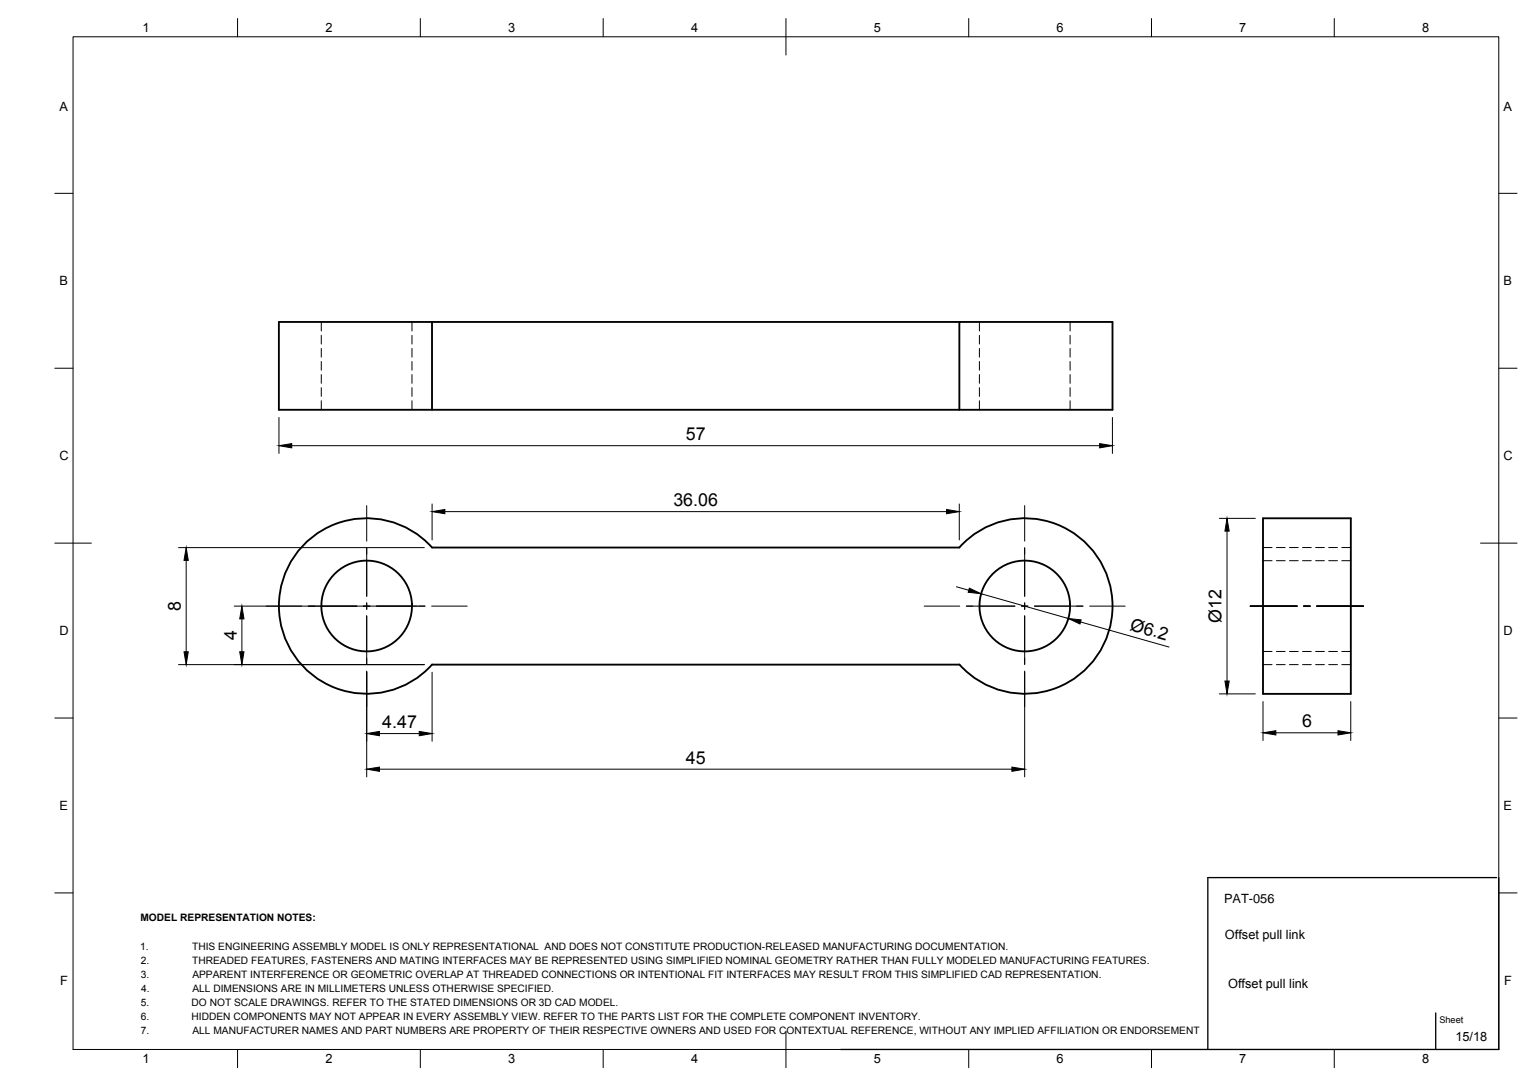
ISO-10303-21;
HEADER;
/* Generated by software containing ST-Developer
 * from STEP Tools, Inc. (www.steptools.com) 
 */

FILE_DESCRIPTION(
/* description */ ('Hook toggle clamp'),
/* implementation_level */ '2;1');

FILE_NAME(
/* name */ 'Offset pull link.step',
/* time_stamp */ '2026-10-27T21:56:56-07:00',
/* author */ (''),
/* organization */ (''),
/* preprocessor_version */ 'ST-DEVELOPER v20.2',
/* originating_system */ 'Autodesk Translation Framework v15.17.0.0',
/* authorisation */ '');

FILE_SCHEMA (('AUTOMOTIVE_DESIGN { 1 0 10303 214 3 1 1 }'));
ENDSEC;

DATA;
#10=MECHANICAL_DESIGN_GEOMETRIC_PRESENTATION_REPRESENTATION('',(#197),#5458);
#163=SHAPE_REPRESENTATION_RELATIONSHIP('SRR','None',#5546,#180);
#180=ADVANCED_BREP_SHAPE_REPRESENTATION('',(#213),#5448);
#197=STYLED_ITEM('',(#5703),#213);
#213=MANIFOLD_SOLID_BREP('Body1',#2979);
#255=FACE_BOUND('',#707,.T.);
#256=FACE_BOUND('',#708,.T.);
#257=FACE_BOUND('',#712,.T.);
#258=FACE_BOUND('',#713,.T.);
#352=PLANE('',#3359);
#353=PLANE('',#3360);
#354=PLANE('',#3362);
#355=PLANE('',#3365);
#496=FACE_OUTER_BOUND('',#702,.T.);
#497=FACE_OUTER_BOUND('',#703,.T.);
#498=FACE_OUTER_BOUND('',#704,.T.);
#499=FACE_OUTER_BOUND('',#705,.T.);
#500=FACE_OUTER_BOUND('',#706,.T.);
#501=FACE_OUTER_BOUND('',#709,.T.);
#502=FACE_OUTER_BOUND('',#710,.T.);
#503=FACE_OUTER_BOUND('',#711,.T.);
#702=EDGE_LOOP('',(#2461,#2462,#2463,#2464));
#703=EDGE_LOOP('',(#2465,#2466,#2467,#2468));
#704=EDGE_LOOP('',(#2469,#2470,#2471,#2472));
#705=EDGE_LOOP('',(#2473,#2474,#2475,#2476));
#706=EDGE_LOOP('',(#2477,#2478,#2479,#2480));
#707=EDGE_LOOP('',(#2481));
#708=EDGE_LOOP('',(#2482));
#709=EDGE_LOOP('',(#2483,#2484,#2485,#2486));
#710=EDGE_LOOP('',(#2487,#2488,#2489,#2490));
#711=EDGE_LOOP('',(#2491,#2492,#2493,#2494));
#712=EDGE_LOOP('',(#2495));
#713=EDGE_LOOP('',(#2496));
#961=LINE('',#4932,#1198);
#962=LINE('',#4938,#1199);
#963=LINE('',#4943,#1200);
#964=LINE('',#4947,#1201);
#965=LINE('',#4951,#1202);
#966=LINE('',#4953,#1203);
#967=LINE('',#4954,#1204);
#968=LINE('',#4957,#1205);
#969=LINE('',#4961,#1206);
#970=LINE('',#4962,#1207);
#1198=VECTOR('',#4029,0.31);
#1199=VECTOR('',#4036,0.31);
#1200=VECTOR('',#4041,1.);
#1201=VECTOR('',#4044,1.);
#1202=VECTOR('',#4049,1.);
#1203=VECTOR('',#4050,1.);
#1204=VECTOR('',#4051,1.);
#1205=VECTOR('',#4054,1.);
#1206=VECTOR('',#4059,1.);
#1207=VECTOR('',#4060,1.);
#1327=CIRCLE('',#3351,0.31);
#1328=CIRCLE('',#3352,0.31);
#1329=CIRCLE('',#3354,0.31);
#1330=CIRCLE('',#3355,0.31);
#1331=CIRCLE('',#3357,0.6);
#1332=CIRCLE('',#3358,0.6);
#1333=CIRCLE('',#3361,0.6);
#1334=CIRCLE('',#3364,0.6);
#1534=VERTEX_POINT('',#4929);
#1535=VERTEX_POINT('',#4931);
#1536=VERTEX_POINT('',#4935);
#1537=VERTEX_POINT('',#4937);
#1538=VERTEX_POINT('',#4941);
#1539=VERTEX_POINT('',#4942);
#1540=VERTEX_POINT('',#4944);
#1541=VERTEX_POINT('',#4946);
#1542=VERTEX_POINT('',#4950);
#1543=VERTEX_POINT('',#4952);
#1544=VERTEX_POINT('',#4956);
#1545=VERTEX_POINT('',#4960);
#1857=EDGE_CURVE('',#1534,#1534,#1327,.T.);
#1858=EDGE_CURVE('',#1534,#1535,#961,.T.);
#1859=EDGE_CURVE('',#1535,#1535,#1328,.T.);
#1860=EDGE_CURVE('',#1536,#1536,#1329,.T.);
#1861=EDGE_CURVE('',#1536,#1537,#962,.T.);
#1862=EDGE_CURVE('',#1537,#1537,#1330,.T.);
#1863=EDGE_CURVE('',#1538,#1539,#963,.T.);
#1864=EDGE_CURVE('',#1540,#1538,#1331,.T.);
#1865=EDGE_CURVE('',#1541,#1540,#964,.T.);
#1866=EDGE_CURVE('',#1541,#1539,#1332,.T.);
#1867=EDGE_CURVE('',#1539,#1542,#965,.T.);
#1868=EDGE_CURVE('',#1543,#1542,#966,.T.);
#1869=EDGE_CURVE('',#1538,#1543,#967,.T.);
#1870=EDGE_CURVE('',#1544,#1541,#968,.T.);
#1871=EDGE_CURVE('',#1542,#1544,#1333,.T.);
#1872=EDGE_CURVE('',#1545,#1540,#969,.T.);
#1873=EDGE_CURVE('',#1544,#1545,#970,.T.);
#1874=EDGE_CURVE('',#1543,#1545,#1334,.T.);
#2461=ORIENTED_EDGE('',*,*,#1857,.F.);
#2462=ORIENTED_EDGE('',*,*,#1858,.T.);
#2463=ORIENTED_EDGE('',*,*,#1859,.F.);
#2464=ORIENTED_EDGE('',*,*,#1858,.F.);
#2465=ORIENTED_EDGE('',*,*,#1860,.F.);
#2466=ORIENTED_EDGE('',*,*,#1861,.T.);
#2467=ORIENTED_EDGE('',*,*,#1862,.F.);
#2468=ORIENTED_EDGE('',*,*,#1861,.F.);
#2469=ORIENTED_EDGE('',*,*,#1863,.F.);
#2470=ORIENTED_EDGE('',*,*,#1864,.F.);
#2471=ORIENTED_EDGE('',*,*,#1865,.F.);
#2472=ORIENTED_EDGE('',*,*,#1866,.T.);
#2473=ORIENTED_EDGE('',*,*,#1863,.T.);
#2474=ORIENTED_EDGE('',*,*,#1867,.T.);
#2475=ORIENTED_EDGE('',*,*,#1868,.F.);
#2476=ORIENTED_EDGE('',*,*,#1869,.F.);
#2477=ORIENTED_EDGE('',*,*,#1866,.F.);
#2478=ORIENTED_EDGE('',*,*,#1870,.F.);
#2479=ORIENTED_EDGE('',*,*,#1871,.F.);
#2480=ORIENTED_EDGE('',*,*,#1867,.F.);
#2481=ORIENTED_EDGE('',*,*,#1857,.T.);
#2482=ORIENTED_EDGE('',*,*,#1860,.T.);
#2483=ORIENTED_EDGE('',*,*,#1865,.T.);
#2484=ORIENTED_EDGE('',*,*,#1872,.F.);
#2485=ORIENTED_EDGE('',*,*,#1873,.F.);
#2486=ORIENTED_EDGE('',*,*,#1870,.T.);
#2487=ORIENTED_EDGE('',*,*,#1868,.T.);
#2488=ORIENTED_EDGE('',*,*,#1871,.T.);
#2489=ORIENTED_EDGE('',*,*,#1873,.T.);
#2490=ORIENTED_EDGE('',*,*,#1874,.F.);
#2491=ORIENTED_EDGE('',*,*,#1869,.T.);
#2492=ORIENTED_EDGE('',*,*,#1874,.T.);
#2493=ORIENTED_EDGE('',*,*,#1872,.T.);
#2494=ORIENTED_EDGE('',*,*,#1864,.T.);
#2495=ORIENTED_EDGE('',*,*,#1859,.T.);
#2496=ORIENTED_EDGE('',*,*,#1862,.T.);
#2774=CYLINDRICAL_SURFACE('',#3350,0.31);
#2775=CYLINDRICAL_SURFACE('',#3353,0.31);
#2776=CYLINDRICAL_SURFACE('',#3356,0.6);
#2777=CYLINDRICAL_SURFACE('',#3363,0.6);
#2900=ADVANCED_FACE('',(#496),#2774,.F.);
#2901=ADVANCED_FACE('',(#497),#2775,.F.);
#2902=ADVANCED_FACE('',(#498),#2776,.T.);
#2903=ADVANCED_FACE('',(#499),#352,.T.);
#2904=ADVANCED_FACE('',(#500,#255,#256),#353,.F.);
#2905=ADVANCED_FACE('',(#501),#354,.T.);
#2906=ADVANCED_FACE('',(#502),#2777,.T.);
#2907=ADVANCED_FACE('',(#503,#257,#258),#355,.T.);
#2979=CLOSED_SHELL('',(#2900,#2901,#2902,#2903,#2904,#2905,#2906,#2907));
#3349=AXIS2_PLACEMENT_3D('',#4927,#4023,#4024);
#3350=AXIS2_PLACEMENT_3D('',#4928,#4025,#4026);
#3351=AXIS2_PLACEMENT_3D('',#4930,#4027,#4028);
#3352=AXIS2_PLACEMENT_3D('',#4933,#4030,#4031);
#3353=AXIS2_PLACEMENT_3D('',#4934,#4032,#4033);
#3354=AXIS2_PLACEMENT_3D('',#4936,#4034,#4035);
#3355=AXIS2_PLACEMENT_3D('',#4939,#4037,#4038);
#3356=AXIS2_PLACEMENT_3D('',#4940,#4039,#4040);
#3357=AXIS2_PLACEMENT_3D('',#4945,#4042,#4043);
#3358=AXIS2_PLACEMENT_3D('',#4948,#4045,#4046);
#3359=AXIS2_PLACEMENT_3D('',#4949,#4047,#4048);
#3360=AXIS2_PLACEMENT_3D('',#4955,#4052,#4053);
#3361=AXIS2_PLACEMENT_3D('',#4958,#4055,#4056);
#3362=AXIS2_PLACEMENT_3D('',#4959,#4057,#4058);
#3363=AXIS2_PLACEMENT_3D('',#4963,#4061,#4062);
#3364=AXIS2_PLACEMENT_3D('',#4964,#4063,#4064);
#3365=AXIS2_PLACEMENT_3D('',#4965,#4065,#4066);
#4023=DIRECTION('axis',(0.,0.,1.));
#4024=DIRECTION('refdir',(1.,0.,0.));
#4025=DIRECTION('center_axis',(0.,1.,0.));
#4026=DIRECTION('ref_axis',(1.,0.,0.));
#4027=DIRECTION('center_axis',(0.,1.,0.));
#4028=DIRECTION('ref_axis',(1.,0.,0.));
#4029=DIRECTION('',(0.,1.,0.));
#4030=DIRECTION('center_axis',(0.,-1.,0.));
#4031=DIRECTION('ref_axis',(1.,0.,0.));
#4032=DIRECTION('center_axis',(0.,1.,0.));
#4033=DIRECTION('ref_axis',(1.,0.,0.));
#4034=DIRECTION('center_axis',(0.,1.,0.));
#4035=DIRECTION('ref_axis',(1.,0.,0.));
#4036=DIRECTION('',(0.,1.,0.));
#4037=DIRECTION('center_axis',(0.,-1.,0.));
#4038=DIRECTION('ref_axis',(1.,0.,0.));
#4039=DIRECTION('center_axis',(0.,1.,0.));
#4040=DIRECTION('ref_axis',(1.,0.,0.));
#4041=DIRECTION('',(0.,-1.,0.));
#4042=DIRECTION('center_axis',(0.,1.,0.));
#4043=DIRECTION('ref_axis',(1.,0.,0.));
#4044=DIRECTION('',(0.,1.,0.));
#4045=DIRECTION('center_axis',(0.,1.,0.));
#4046=DIRECTION('ref_axis',(1.,0.,0.));
#4047=DIRECTION('center_axis',(0.0484198570820323,0.,-0.998827070838669));
#4048=DIRECTION('ref_axis',(-0.998827070838669,0.,-0.0484198570820323));
#4049=DIRECTION('',(-0.998827070838669,0.,-0.0484198570820323));
#4050=DIRECTION('',(0.,-1.,0.));
#4051=DIRECTION('',(-0.998827070838669,0.,-0.0484198570820323));
#4052=DIRECTION('center_axis',(0.,1.,0.));
#4053=DIRECTION('ref_axis',(1.,0.,0.));
#4054=DIRECTION('',(0.998827070838669,0.,0.0484198570820322));
#4055=DIRECTION('center_axis',(0.,1.,0.));
#4056=DIRECTION('ref_axis',(1.,0.,0.));
#4057=DIRECTION('center_axis',(-0.0484198570820322,0.,0.998827070838669));
#4058=DIRECTION('ref_axis',(0.998827070838669,0.,0.0484198570820322));
#4059=DIRECTION('',(0.998827070838669,0.,0.0484198570820322));
#4060=DIRECTION('',(0.,1.,0.));
#4061=DIRECTION('center_axis',(0.,1.,0.));
#4062=DIRECTION('ref_axis',(-0.998827070838669,0.,-0.0484198570820321));
#4063=DIRECTION('center_axis',(0.,1.,0.));
#4064=DIRECTION('ref_axis',(1.,0.,0.));
#4065=DIRECTION('center_axis',(0.,1.,0.));
#4066=DIRECTION('ref_axis',(1.,0.,0.));
#4927=CARTESIAN_POINT('',(0.,0.,0.));
#4928=CARTESIAN_POINT('Origin',(-2.49048674522936,1.,2.28211064313086));
#4929=CARTESIAN_POINT('',(-2.80048674522936,1.1,2.28211064313086));
#4930=CARTESIAN_POINT('Origin',(-2.49048674522936,1.1,2.28211064313086));
#4931=CARTESIAN_POINT('',(-2.80048674522936,1.7,2.28211064313086));
#4932=CARTESIAN_POINT('',(-2.80048674522936,1.,2.28211064313086));
#4933=CARTESIAN_POINT('Origin',(-2.49048674522936,1.7,2.28211064313086));
#4934=CARTESIAN_POINT('Origin',(2.00423507354465,1.,2.5));
#4935=CARTESIAN_POINT('',(1.69423507354465,1.1,2.5));
#4936=CARTESIAN_POINT('Origin',(2.00423507354465,1.1,2.5));
#4937=CARTESIAN_POINT('',(1.69423507354465,1.7,2.5));
#4938=CARTESIAN_POINT('',(1.69423507354465,1.,2.5));
#4939=CARTESIAN_POINT('Origin',(2.00423507354465,1.7,2.5));
#4940=CARTESIAN_POINT('Origin',(2.00423507354465,1.1,2.5));
#4941=CARTESIAN_POINT('',(1.57691397074501,1.7,2.07881515328528));
#4942=CARTESIAN_POINT('',(1.57691397074501,1.1,2.07881515328528));
#4943=CARTESIAN_POINT('',(1.57691397074501,1.1,2.07881515328528));
#4944=CARTESIAN_POINT('',(1.53817808507938,1.7,2.87787680995622));
#4945=CARTESIAN_POINT('Origin',(2.00423507354465,1.7,2.5));
#4946=CARTESIAN_POINT('',(1.53817808507938,1.1,2.87787680995622));
#4947=CARTESIAN_POINT('',(1.53817808507938,1.1,2.87787680995622));
#4948=CARTESIAN_POINT('Origin',(2.00423507354465,1.1,2.5));
#4949=CARTESIAN_POINT('Origin',(2.02360301637746,1.1,2.10046917166453));
#4950=CARTESIAN_POINT('',(-2.0244297567641,1.1,1.90423383317464));
#4951=CARTESIAN_POINT('',(2.02360301637746,1.1,2.10046917166453));
#4952=CARTESIAN_POINT('',(-2.0244297567641,1.7,1.90423383317464));
#4953=CARTESIAN_POINT('',(-2.0244297567641,1.1,1.90423383317464));
#4954=CARTESIAN_POINT('',(2.02360301637746,1.7,2.10046917166453));
#4955=CARTESIAN_POINT('Origin',(-2.49048674522936,1.1,2.28211064313086));
#4956=CARTESIAN_POINT('',(-2.06316564242972,1.1,2.70329548984557));
#4957=CARTESIAN_POINT('',(-2.50985468806218,1.1,2.68164147146632));
#4958=CARTESIAN_POINT('Origin',(-2.49048674522936,1.1,2.28211064313086));
#4959=CARTESIAN_POINT('Origin',(-2.50985468806218,1.1,2.68164147146632));
#4960=CARTESIAN_POINT('',(-2.06316564242972,1.7,2.70329548984557));
#4961=CARTESIAN_POINT('',(-2.50985468806218,1.7,2.68164147146632));
#4962=CARTESIAN_POINT('',(-2.06316564242972,1.1,2.70329548984557));
#4963=CARTESIAN_POINT('Origin',(-2.49048674522936,1.1,2.28211064313086));
#4964=CARTESIAN_POINT('Origin',(-2.49048674522936,1.7,2.28211064313086));
#4965=CARTESIAN_POINT('Origin',(-2.49048674522936,1.7,2.28211064313086));
#5425=UNCERTAINTY_MEASURE_WITH_UNIT(LENGTH_MEASURE(0.001),#5459,
'DISTANCE_ACCURACY_VALUE',
'Maximum model space distance between geometric entities at asserted c
onnectivities');
#5435=UNCERTAINTY_MEASURE_WITH_UNIT(LENGTH_MEASURE(0.001),#5459,
'DISTANCE_ACCURACY_VALUE',
'Maximum model space distance between geometric entities at asserted c
onnectivities');
#5448=(
GEOMETRIC_REPRESENTATION_CONTEXT(3)
GLOBAL_UNCERTAINTY_ASSIGNED_CONTEXT((#5425))
GLOBAL_UNIT_ASSIGNED_CONTEXT((#5459,#5461,#5462))
REPRESENTATION_CONTEXT('','3D')
);
#5458=(
GEOMETRIC_REPRESENTATION_CONTEXT(3)
GLOBAL_UNCERTAINTY_ASSIGNED_CONTEXT((#5435))
GLOBAL_UNIT_ASSIGNED_CONTEXT((#5459,#5461,#5462))
REPRESENTATION_CONTEXT('','3D')
);
#5459=(
LENGTH_UNIT()
NAMED_UNIT(*)
SI_UNIT(.CENTI.,.METRE.)
);
#5461=(
NAMED_UNIT(*)
PLANE_ANGLE_UNIT()
SI_UNIT($,.RADIAN.)
);
#5462=(
NAMED_UNIT(*)
SI_UNIT($,.STERADIAN.)
SOLID_ANGLE_UNIT()
);
#5475=SHAPE_DEFINITION_REPRESENTATION(#5497,#5546);
#5497=PRODUCT_DEFINITION_SHAPE('',$,#5569);
#5546=SHAPE_REPRESENTATION('',(#3349),#5448);
#5556=PRODUCT_DEFINITION_CONTEXT('part definition',#5624,'design');
#5569=PRODUCT_DEFINITION('Offset pull link','Offset pull link',#5591,#5556);
#5591=PRODUCT_DEFINITION_FORMATION('',$,#5638);
#5624=APPLICATION_CONTEXT(
'Core Data for Automotive Mechanical Design Process');
#5625=PRODUCT_CONTEXT('part definition',#5624,'mechanical');
#5638=PRODUCT('Offset pull link','Offset pull link','Offset pull link',
(#5625));
#5697=COLOUR_RGB('Light Blue',0.38,0.62,0.78);
#5698=FILL_AREA_STYLE_COLOUR('',#5697);
#5699=FILL_AREA_STYLE('',(#5698));
#5700=SURFACE_STYLE_FILL_AREA(#5699);
#5701=SURFACE_SIDE_STYLE('',(#5700));
#5702=SURFACE_STYLE_USAGE(.BOTH.,#5701);
#5703=PRESENTATION_STYLE_ASSIGNMENT((#5702));
ENDSEC;
END-ISO-10303-21;
